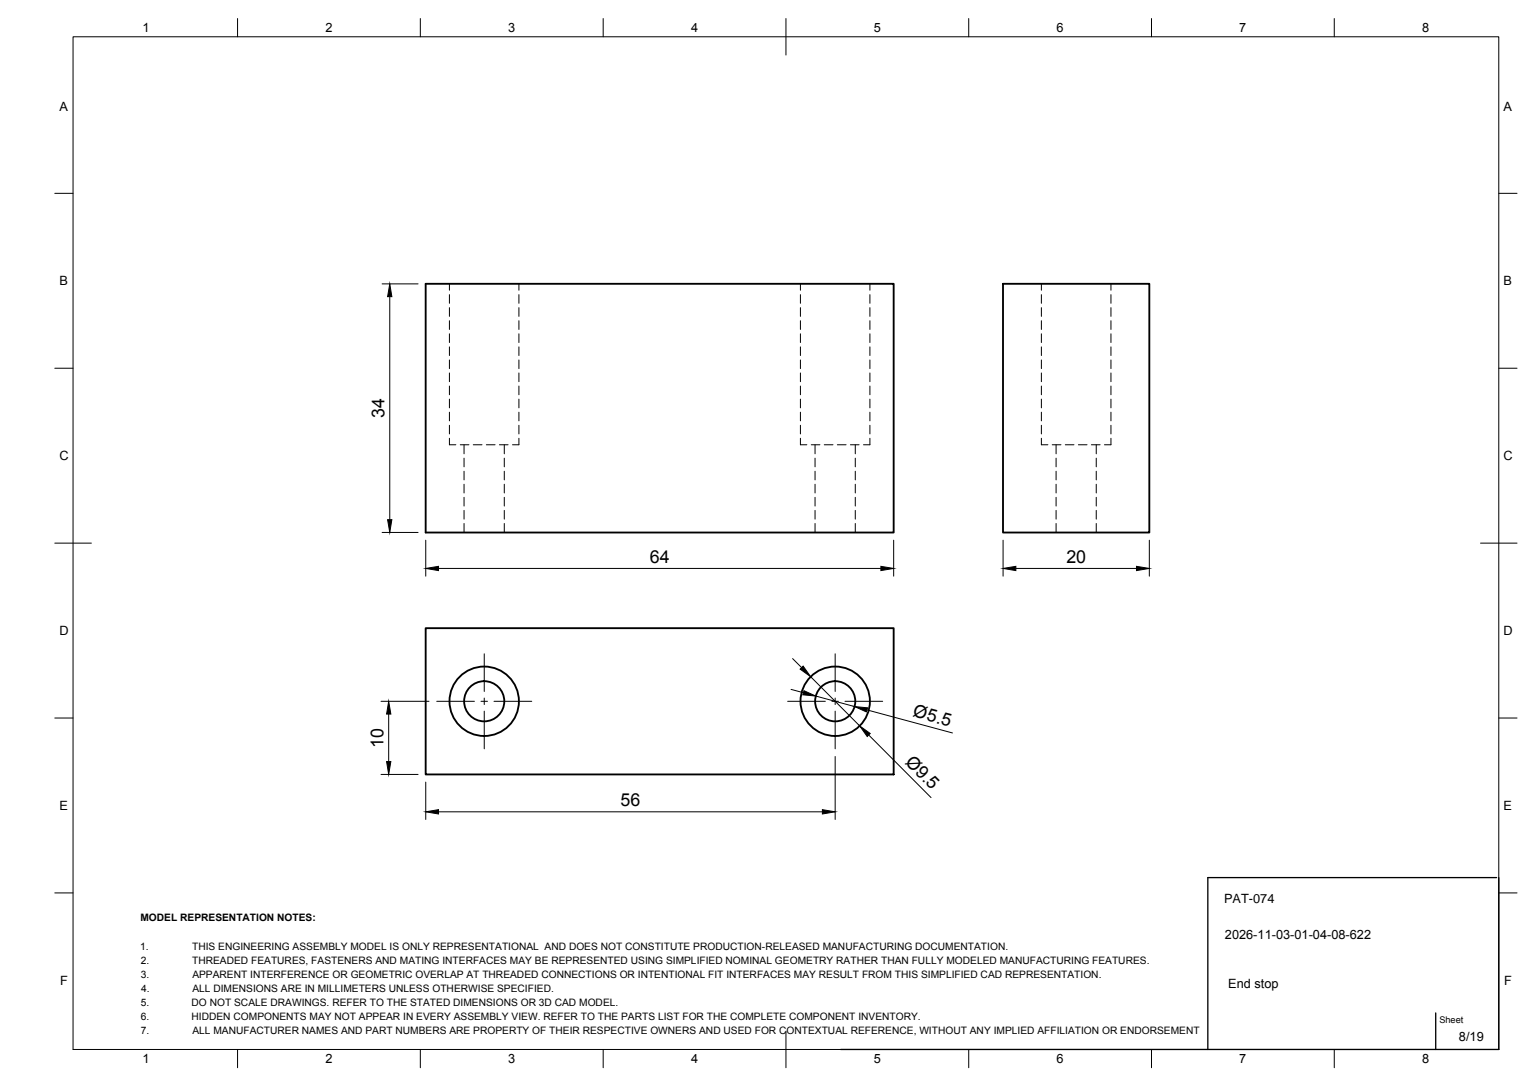
ISO-10303-21;
HEADER;
/* Generated by software containing ST-Developer
 * from STEP Tools, Inc. (www.steptools.com) 
 */

FILE_DESCRIPTION(
/* description */ ('Manual rail carriage with stops'),
/* implementation_level */ '2;1');

FILE_NAME(
/* name */ 'End stop.step',
/* time_stamp */ '2026-10-27T18:54:27-07:00',
/* author */ (''),
/* organization */ (''),
/* preprocessor_version */ 'ST-DEVELOPER v20.2',
/* originating_system */ 'Autodesk Translation Framework v15.17.0.0',
/* authorisation */ '');

FILE_SCHEMA (('AUTOMOTIVE_DESIGN { 1 0 10303 214 3 1 1 }'));
ENDSEC;

DATA;
#10=MECHANICAL_DESIGN_GEOMETRIC_PRESENTATION_REPRESENTATION('',(#279),#8499);
#243=SHAPE_REPRESENTATION_RELATIONSHIP('SRR','None',#8606,#261);
#261=ADVANCED_BREP_SHAPE_REPRESENTATION('',(#295),#8485);
#279=STYLED_ITEM('',(#8781),#295);
#295=MANIFOLD_SOLID_BREP('Body1',#4949);
#350=FACE_BOUND('',#1029,.T.);
#351=FACE_BOUND('',#1032,.T.);
#352=FACE_BOUND('',#1040,.T.);
#353=FACE_BOUND('',#1041,.T.);
#354=FACE_BOUND('',#1043,.T.);
#355=FACE_BOUND('',#1044,.T.);
#485=PLANE('',#5381);
#486=PLANE('',#5386);
#487=PLANE('',#5392);
#488=PLANE('',#5393);
#489=PLANE('',#5394);
#490=PLANE('',#5395);
#491=PLANE('',#5396);
#492=PLANE('',#5397);
#717=FACE_OUTER_BOUND('',#1027,.T.);
#718=FACE_OUTER_BOUND('',#1028,.T.);
#719=FACE_OUTER_BOUND('',#1030,.T.);
#720=FACE_OUTER_BOUND('',#1031,.T.);
#721=FACE_OUTER_BOUND('',#1033,.T.);
#722=FACE_OUTER_BOUND('',#1034,.T.);
#723=FACE_OUTER_BOUND('',#1035,.T.);
#724=FACE_OUTER_BOUND('',#1036,.T.);
#725=FACE_OUTER_BOUND('',#1037,.T.);
#726=FACE_OUTER_BOUND('',#1038,.T.);
#727=FACE_OUTER_BOUND('',#1039,.T.);
#728=FACE_OUTER_BOUND('',#1042,.T.);
#1027=EDGE_LOOP('',(#4060,#4061,#4062,#4063));
#1028=EDGE_LOOP('',(#4064));
#1029=EDGE_LOOP('',(#4065));
#1030=EDGE_LOOP('',(#4066,#4067,#4068,#4069));
#1031=EDGE_LOOP('',(#4070));
#1032=EDGE_LOOP('',(#4071));
#1033=EDGE_LOOP('',(#4072,#4073,#4074,#4075));
#1034=EDGE_LOOP('',(#4076,#4077,#4078,#4079));
#1035=EDGE_LOOP('',(#4080,#4081,#4082,#4083));
#1036=EDGE_LOOP('',(#4084,#4085,#4086,#4087));
#1037=EDGE_LOOP('',(#4088,#4089,#4090,#4091));
#1038=EDGE_LOOP('',(#4092,#4093,#4094,#4095));
#1039=EDGE_LOOP('',(#4096,#4097,#4098,#4099));
#1040=EDGE_LOOP('',(#4100));
#1041=EDGE_LOOP('',(#4101));
#1042=EDGE_LOOP('',(#4102,#4103,#4104,#4105));
#1043=EDGE_LOOP('',(#4106));
#1044=EDGE_LOOP('',(#4107));
#1465=LINE('',#7803,#1965);
#1466=LINE('',#7812,#1966);
#1467=LINE('',#7820,#1967);
#1468=LINE('',#7824,#1968);
#1469=LINE('',#7828,#1969);
#1470=LINE('',#7830,#1970);
#1471=LINE('',#7832,#1971);
#1472=LINE('',#7833,#1972);
#1473=LINE('',#7836,#1973);
#1474=LINE('',#7838,#1974);
#1475=LINE('',#7839,#1975);
#1476=LINE('',#7842,#1976);
#1477=LINE('',#7844,#1977);
#1478=LINE('',#7845,#1978);
#1479=LINE('',#7847,#1979);
#1480=LINE('',#7848,#1980);
#1965=VECTOR('',#6350,0.475);
#1966=VECTOR('',#6361,0.475);
#1967=VECTOR('',#6372,0.275);
#1968=VECTOR('',#6377,0.275);
#1969=VECTOR('',#6380,1.);
#1970=VECTOR('',#6381,1.);
#1971=VECTOR('',#6382,1.);
#1972=VECTOR('',#6383,1.);
#1973=VECTOR('',#6386,1.);
#1974=VECTOR('',#6387,1.);
#1975=VECTOR('',#6388,1.);
#1976=VECTOR('',#6391,1.);
#1977=VECTOR('',#6392,1.);
#1978=VECTOR('',#6393,1.);
#1979=VECTOR('',#6396,1.);
#1980=VECTOR('',#6397,1.);
#2247=CIRCLE('',#5379,0.475);
#2248=CIRCLE('',#5380,0.475);
#2249=CIRCLE('',#5382,0.275);
#2250=CIRCLE('',#5384,0.475);
#2251=CIRCLE('',#5385,0.475);
#2252=CIRCLE('',#5387,0.275);
#2253=CIRCLE('',#5389,0.275);
#2254=CIRCLE('',#5391,0.275);
#2543=VERTEX_POINT('',#7800);
#2544=VERTEX_POINT('',#7802);
#2545=VERTEX_POINT('',#7806);
#2546=VERTEX_POINT('',#7809);
#2547=VERTEX_POINT('',#7811);
#2548=VERTEX_POINT('',#7815);
#2549=VERTEX_POINT('',#7818);
#2550=VERTEX_POINT('',#7822);
#2551=VERTEX_POINT('',#7826);
#2552=VERTEX_POINT('',#7827);
#2553=VERTEX_POINT('',#7829);
#2554=VERTEX_POINT('',#7831);
#2555=VERTEX_POINT('',#7835);
#2556=VERTEX_POINT('',#7837);
#2557=VERTEX_POINT('',#7841);
#2558=VERTEX_POINT('',#7843);
#3078=EDGE_CURVE('',#2543,#2543,#2247,.T.);
#3079=EDGE_CURVE('',#2543,#2544,#1465,.T.);
#3080=EDGE_CURVE('',#2544,#2544,#2248,.T.);
#3081=EDGE_CURVE('',#2545,#2545,#2249,.T.);
#3082=EDGE_CURVE('',#2546,#2546,#2250,.T.);
#3083=EDGE_CURVE('',#2546,#2547,#1466,.T.);
#3084=EDGE_CURVE('',#2547,#2547,#2251,.T.);
#3085=EDGE_CURVE('',#2548,#2548,#2252,.T.);
#3086=EDGE_CURVE('',#2549,#2549,#2253,.T.);
#3087=EDGE_CURVE('',#2549,#2545,#1467,.T.);
#3088=EDGE_CURVE('',#2550,#2550,#2254,.T.);
#3089=EDGE_CURVE('',#2550,#2548,#1468,.T.);
#3090=EDGE_CURVE('',#2551,#2552,#1469,.T.);
#3091=EDGE_CURVE('',#2552,#2553,#1470,.T.);
#3092=EDGE_CURVE('',#2554,#2553,#1471,.T.);
#3093=EDGE_CURVE('',#2551,#2554,#1472,.T.);
#3094=EDGE_CURVE('',#2555,#2551,#1473,.T.);
#3095=EDGE_CURVE('',#2556,#2554,#1474,.T.);
#3096=EDGE_CURVE('',#2555,#2556,#1475,.T.);
#3097=EDGE_CURVE('',#2557,#2555,#1476,.T.);
#3098=EDGE_CURVE('',#2558,#2556,#1477,.T.);
#3099=EDGE_CURVE('',#2557,#2558,#1478,.T.);
#3100=EDGE_CURVE('',#2552,#2557,#1479,.T.);
#3101=EDGE_CURVE('',#2553,#2558,#1480,.T.);
#4060=ORIENTED_EDGE('',*,*,#3078,.F.);
#4061=ORIENTED_EDGE('',*,*,#3079,.T.);
#4062=ORIENTED_EDGE('',*,*,#3080,.F.);
#4063=ORIENTED_EDGE('',*,*,#3079,.F.);
#4064=ORIENTED_EDGE('',*,*,#3078,.T.);
#4065=ORIENTED_EDGE('',*,*,#3081,.F.);
#4066=ORIENTED_EDGE('',*,*,#3082,.F.);
#4067=ORIENTED_EDGE('',*,*,#3083,.T.);
#4068=ORIENTED_EDGE('',*,*,#3084,.F.);
#4069=ORIENTED_EDGE('',*,*,#3083,.F.);
#4070=ORIENTED_EDGE('',*,*,#3082,.T.);
#4071=ORIENTED_EDGE('',*,*,#3085,.F.);
#4072=ORIENTED_EDGE('',*,*,#3086,.F.);
#4073=ORIENTED_EDGE('',*,*,#3087,.T.);
#4074=ORIENTED_EDGE('',*,*,#3081,.T.);
#4075=ORIENTED_EDGE('',*,*,#3087,.F.);
#4076=ORIENTED_EDGE('',*,*,#3088,.F.);
#4077=ORIENTED_EDGE('',*,*,#3089,.T.);
#4078=ORIENTED_EDGE('',*,*,#3085,.T.);
#4079=ORIENTED_EDGE('',*,*,#3089,.F.);
#4080=ORIENTED_EDGE('',*,*,#3090,.T.);
#4081=ORIENTED_EDGE('',*,*,#3091,.T.);
#4082=ORIENTED_EDGE('',*,*,#3092,.F.);
#4083=ORIENTED_EDGE('',*,*,#3093,.F.);
#4084=ORIENTED_EDGE('',*,*,#3094,.T.);
#4085=ORIENTED_EDGE('',*,*,#3093,.T.);
#4086=ORIENTED_EDGE('',*,*,#3095,.F.);
#4087=ORIENTED_EDGE('',*,*,#3096,.F.);
#4088=ORIENTED_EDGE('',*,*,#3097,.T.);
#4089=ORIENTED_EDGE('',*,*,#3096,.T.);
#4090=ORIENTED_EDGE('',*,*,#3098,.F.);
#4091=ORIENTED_EDGE('',*,*,#3099,.F.);
#4092=ORIENTED_EDGE('',*,*,#3100,.T.);
#4093=ORIENTED_EDGE('',*,*,#3099,.T.);
#4094=ORIENTED_EDGE('',*,*,#3101,.F.);
#4095=ORIENTED_EDGE('',*,*,#3091,.F.);
#4096=ORIENTED_EDGE('',*,*,#3101,.T.);
#4097=ORIENTED_EDGE('',*,*,#3098,.T.);
#4098=ORIENTED_EDGE('',*,*,#3095,.T.);
#4099=ORIENTED_EDGE('',*,*,#3092,.T.);
#4100=ORIENTED_EDGE('',*,*,#3080,.T.);
#4101=ORIENTED_EDGE('',*,*,#3084,.T.);
#4102=ORIENTED_EDGE('',*,*,#3100,.F.);
#4103=ORIENTED_EDGE('',*,*,#3090,.F.);
#4104=ORIENTED_EDGE('',*,*,#3094,.F.);
#4105=ORIENTED_EDGE('',*,*,#3097,.F.);
#4106=ORIENTED_EDGE('',*,*,#3086,.T.);
#4107=ORIENTED_EDGE('',*,*,#3088,.T.);
#4652=CYLINDRICAL_SURFACE('',#5378,0.475);
#4653=CYLINDRICAL_SURFACE('',#5383,0.475);
#4654=CYLINDRICAL_SURFACE('',#5388,0.275);
#4655=CYLINDRICAL_SURFACE('',#5390,0.275);
#4816=ADVANCED_FACE('',(#717),#4652,.F.);
#4817=ADVANCED_FACE('',(#718,#350),#485,.T.);
#4818=ADVANCED_FACE('',(#719),#4653,.F.);
#4819=ADVANCED_FACE('',(#720,#351),#486,.T.);
#4820=ADVANCED_FACE('',(#721),#4654,.F.);
#4821=ADVANCED_FACE('',(#722),#4655,.F.);
#4822=ADVANCED_FACE('',(#723),#487,.T.);
#4823=ADVANCED_FACE('',(#724),#488,.T.);
#4824=ADVANCED_FACE('',(#725),#489,.T.);
#4825=ADVANCED_FACE('',(#726),#490,.T.);
#4826=ADVANCED_FACE('',(#727,#352,#353),#491,.T.);
#4827=ADVANCED_FACE('',(#728,#354,#355),#492,.F.);
#4949=CLOSED_SHELL('',(#4816,#4817,#4818,#4819,#4820,#4821,#4822,#4823,
#4824,#4825,#4826,#4827));
#5377=AXIS2_PLACEMENT_3D('',#7798,#6344,#6345);
#5378=AXIS2_PLACEMENT_3D('',#7799,#6346,#6347);
#5379=AXIS2_PLACEMENT_3D('',#7801,#6348,#6349);
#5380=AXIS2_PLACEMENT_3D('',#7804,#6351,#6352);
#5381=AXIS2_PLACEMENT_3D('',#7805,#6353,#6354);
#5382=AXIS2_PLACEMENT_3D('',#7807,#6355,#6356);
#5383=AXIS2_PLACEMENT_3D('',#7808,#6357,#6358);
#5384=AXIS2_PLACEMENT_3D('',#7810,#6359,#6360);
#5385=AXIS2_PLACEMENT_3D('',#7813,#6362,#6363);
#5386=AXIS2_PLACEMENT_3D('',#7814,#6364,#6365);
#5387=AXIS2_PLACEMENT_3D('',#7816,#6366,#6367);
#5388=AXIS2_PLACEMENT_3D('',#7817,#6368,#6369);
#5389=AXIS2_PLACEMENT_3D('',#7819,#6370,#6371);
#5390=AXIS2_PLACEMENT_3D('',#7821,#6373,#6374);
#5391=AXIS2_PLACEMENT_3D('',#7823,#6375,#6376);
#5392=AXIS2_PLACEMENT_3D('',#7825,#6378,#6379);
#5393=AXIS2_PLACEMENT_3D('',#7834,#6384,#6385);
#5394=AXIS2_PLACEMENT_3D('',#7840,#6389,#6390);
#5395=AXIS2_PLACEMENT_3D('',#7846,#6394,#6395);
#5396=AXIS2_PLACEMENT_3D('',#7849,#6398,#6399);
#5397=AXIS2_PLACEMENT_3D('',#7850,#6400,#6401);
#6344=DIRECTION('axis',(0.,0.,1.));
#6345=DIRECTION('refdir',(1.,0.,0.));
#6346=DIRECTION('center_axis',(0.,0.,1.));
#6347=DIRECTION('ref_axis',(1.,0.,0.));
#6348=DIRECTION('center_axis',(0.,0.,1.));
#6349=DIRECTION('ref_axis',(1.,0.,0.));
#6350=DIRECTION('',(0.,0.,1.));
#6351=DIRECTION('center_axis',(0.,0.,-1.));
#6352=DIRECTION('ref_axis',(1.,0.,0.));
#6353=DIRECTION('center_axis',(0.,0.,1.));
#6354=DIRECTION('ref_axis',(1.,0.,0.));
#6355=DIRECTION('center_axis',(0.,0.,1.));
#6356=DIRECTION('ref_axis',(1.,0.,0.));
#6357=DIRECTION('center_axis',(0.,0.,1.));
#6358=DIRECTION('ref_axis',(1.,0.,0.));
#6359=DIRECTION('center_axis',(0.,0.,1.));
#6360=DIRECTION('ref_axis',(1.,0.,0.));
#6361=DIRECTION('',(0.,0.,1.));
#6362=DIRECTION('center_axis',(0.,0.,-1.));
#6363=DIRECTION('ref_axis',(1.,0.,0.));
#6364=DIRECTION('center_axis',(0.,0.,1.));
#6365=DIRECTION('ref_axis',(1.,0.,0.));
#6366=DIRECTION('center_axis',(0.,0.,1.));
#6367=DIRECTION('ref_axis',(1.,0.,0.));
#6368=DIRECTION('center_axis',(0.,0.,1.));
#6369=DIRECTION('ref_axis',(1.,0.,0.));
#6370=DIRECTION('center_axis',(0.,0.,1.));
#6371=DIRECTION('ref_axis',(1.,0.,0.));
#6372=DIRECTION('',(0.,0.,1.));
#6373=DIRECTION('center_axis',(0.,0.,1.));
#6374=DIRECTION('ref_axis',(1.,0.,0.));
#6375=DIRECTION('center_axis',(0.,0.,1.));
#6376=DIRECTION('ref_axis',(1.,0.,0.));
#6377=DIRECTION('',(0.,0.,1.));
#6378=DIRECTION('center_axis',(0.,1.,0.));
#6379=DIRECTION('ref_axis',(-1.,0.,0.));
#6380=DIRECTION('',(-1.,0.,0.));
#6381=DIRECTION('',(0.,0.,1.));
#6382=DIRECTION('',(-1.,0.,0.));
#6383=DIRECTION('',(0.,0.,1.));
#6384=DIRECTION('center_axis',(1.,0.,0.));
#6385=DIRECTION('ref_axis',(0.,1.,0.));
#6386=DIRECTION('',(0.,1.,0.));
#6387=DIRECTION('',(0.,1.,0.));
#6388=DIRECTION('',(0.,0.,1.));
#6389=DIRECTION('center_axis',(0.,-1.,0.));
#6390=DIRECTION('ref_axis',(1.,0.,0.));
#6391=DIRECTION('',(1.,0.,0.));
#6392=DIRECTION('',(1.,0.,0.));
#6393=DIRECTION('',(0.,0.,1.));
#6394=DIRECTION('center_axis',(-1.,0.,0.));
#6395=DIRECTION('ref_axis',(0.,-1.,0.));
#6396=DIRECTION('',(0.,-1.,0.));
#6397=DIRECTION('',(0.,-1.,0.));
#6398=DIRECTION('center_axis',(0.,0.,1.));
#6399=DIRECTION('ref_axis',(1.,0.,0.));
#6400=DIRECTION('center_axis',(0.,0.,1.));
#6401=DIRECTION('ref_axis',(1.,0.,0.));
#7798=CARTESIAN_POINT('',(0.,0.,0.));
#7799=CARTESIAN_POINT('Origin',(-1.,-2.4,4.));
#7800=CARTESIAN_POINT('',(-1.475,-2.4,4.));
#7801=CARTESIAN_POINT('Origin',(-1.,-2.4,4.));
#7802=CARTESIAN_POINT('',(-1.475,-2.4,6.2));
#7803=CARTESIAN_POINT('',(-1.475,-2.4,4.));
#7804=CARTESIAN_POINT('Origin',(-1.,-2.4,6.2));
#7805=CARTESIAN_POINT('Origin',(-1.,-2.4,4.));
#7806=CARTESIAN_POINT('',(-1.275,-2.4,4.));
#7807=CARTESIAN_POINT('Origin',(-1.,-2.4,4.));
#7808=CARTESIAN_POINT('Origin',(-1.,2.4,4.));
#7809=CARTESIAN_POINT('',(-1.475,2.4,4.));
#7810=CARTESIAN_POINT('Origin',(-1.,2.4,4.));
#7811=CARTESIAN_POINT('',(-1.475,2.4,6.2));
#7812=CARTESIAN_POINT('',(-1.475,2.4,4.));
#7813=CARTESIAN_POINT('Origin',(-1.,2.4,6.2));
#7814=CARTESIAN_POINT('Origin',(-1.,2.4,4.));
#7815=CARTESIAN_POINT('',(-1.275,2.4,4.));
#7816=CARTESIAN_POINT('Origin',(-1.,2.4,4.));
#7817=CARTESIAN_POINT('Origin',(-1.,-2.4,2.7));
#7818=CARTESIAN_POINT('',(-1.275,-2.4,2.8));
#7819=CARTESIAN_POINT('Origin',(-1.,-2.4,2.8));
#7820=CARTESIAN_POINT('',(-1.275,-2.4,2.7));
#7821=CARTESIAN_POINT('Origin',(-1.,2.4,2.7));
#7822=CARTESIAN_POINT('',(-1.275,2.4,2.8));
#7823=CARTESIAN_POINT('Origin',(-1.,2.4,2.8));
#7824=CARTESIAN_POINT('',(-1.275,2.4,2.7));
#7825=CARTESIAN_POINT('Origin',(0.,3.2,2.8));
#7826=CARTESIAN_POINT('',(0.,3.2,2.8));
#7827=CARTESIAN_POINT('',(-2.,3.2,2.8));
#7828=CARTESIAN_POINT('',(0.,3.2,2.8));
#7829=CARTESIAN_POINT('',(-2.,3.2,6.2));
#7830=CARTESIAN_POINT('',(-2.,3.2,2.8));
#7831=CARTESIAN_POINT('',(0.,3.2,6.2));
#7832=CARTESIAN_POINT('',(0.,3.2,6.2));
#7833=CARTESIAN_POINT('',(0.,3.2,2.8));
#7834=CARTESIAN_POINT('Origin',(0.,-3.2,2.8));
#7835=CARTESIAN_POINT('',(0.,-3.2,2.8));
#7836=CARTESIAN_POINT('',(0.,-3.2,2.8));
#7837=CARTESIAN_POINT('',(0.,-3.2,6.2));
#7838=CARTESIAN_POINT('',(0.,-3.2,6.2));
#7839=CARTESIAN_POINT('',(0.,-3.2,2.8));
#7840=CARTESIAN_POINT('Origin',(-2.,-3.2,2.8));
#7841=CARTESIAN_POINT('',(-2.,-3.2,2.8));
#7842=CARTESIAN_POINT('',(-2.,-3.2,2.8));
#7843=CARTESIAN_POINT('',(-2.,-3.2,6.2));
#7844=CARTESIAN_POINT('',(-2.,-3.2,6.2));
#7845=CARTESIAN_POINT('',(-2.,-3.2,2.8));
#7846=CARTESIAN_POINT('Origin',(-2.,3.2,2.8));
#7847=CARTESIAN_POINT('',(-2.,3.2,2.8));
#7848=CARTESIAN_POINT('',(-2.,3.2,6.2));
#7849=CARTESIAN_POINT('Origin',(-1.,0.,6.2));
#7850=CARTESIAN_POINT('Origin',(-1.,0.,2.8));
#8462=UNCERTAINTY_MEASURE_WITH_UNIT(LENGTH_MEASURE(0.001),#8500,
'DISTANCE_ACCURACY_VALUE',
'Maximum model space distance between geometric entities at asserted c
onnectivities');
#8476=UNCERTAINTY_MEASURE_WITH_UNIT(LENGTH_MEASURE(0.001),#8500,
'DISTANCE_ACCURACY_VALUE',
'Maximum model space distance between geometric entities at asserted c
onnectivities');
#8485=(
GEOMETRIC_REPRESENTATION_CONTEXT(3)
GLOBAL_UNCERTAINTY_ASSIGNED_CONTEXT((#8462))
GLOBAL_UNIT_ASSIGNED_CONTEXT((#8500,#8502,#8503))
REPRESENTATION_CONTEXT('','3D')
);
#8499=(
GEOMETRIC_REPRESENTATION_CONTEXT(3)
GLOBAL_UNCERTAINTY_ASSIGNED_CONTEXT((#8476))
GLOBAL_UNIT_ASSIGNED_CONTEXT((#8500,#8502,#8503))
REPRESENTATION_CONTEXT('','3D')
);
#8500=(
LENGTH_UNIT()
NAMED_UNIT(*)
SI_UNIT(.CENTI.,.METRE.)
);
#8502=(
NAMED_UNIT(*)
PLANE_ANGLE_UNIT()
SI_UNIT($,.RADIAN.)
);
#8503=(
NAMED_UNIT(*)
SI_UNIT($,.STERADIAN.)
SOLID_ANGLE_UNIT()
);
#8512=SHAPE_DEFINITION_REPRESENTATION(#8534,#8606);
#8534=PRODUCT_DEFINITION_SHAPE('',$,#8629);
#8606=SHAPE_REPRESENTATION('',(#5377),#8485);
#8620=PRODUCT_DEFINITION_CONTEXT('part definition',#8688,'design');
#8629=PRODUCT_DEFINITION('End stop','End stop',#8651,#8620);
#8651=PRODUCT_DEFINITION_FORMATION('',$,#8698);
#8688=APPLICATION_CONTEXT(
'Core Data for Automotive Mechanical Design Process');
#8689=PRODUCT_CONTEXT('part definition',#8688,'mechanical');
#8698=PRODUCT('End stop','End stop','End stop',(#8689));
#8775=COLOUR_RGB('Sky Blue',0.24,0.69,0.87);
#8776=FILL_AREA_STYLE_COLOUR('',#8775);
#8777=FILL_AREA_STYLE('',(#8776));
#8778=SURFACE_STYLE_FILL_AREA(#8777);
#8779=SURFACE_SIDE_STYLE('',(#8778));
#8780=SURFACE_STYLE_USAGE(.BOTH.,#8779);
#8781=PRESENTATION_STYLE_ASSIGNMENT((#8780));
ENDSEC;
END-ISO-10303-21;
